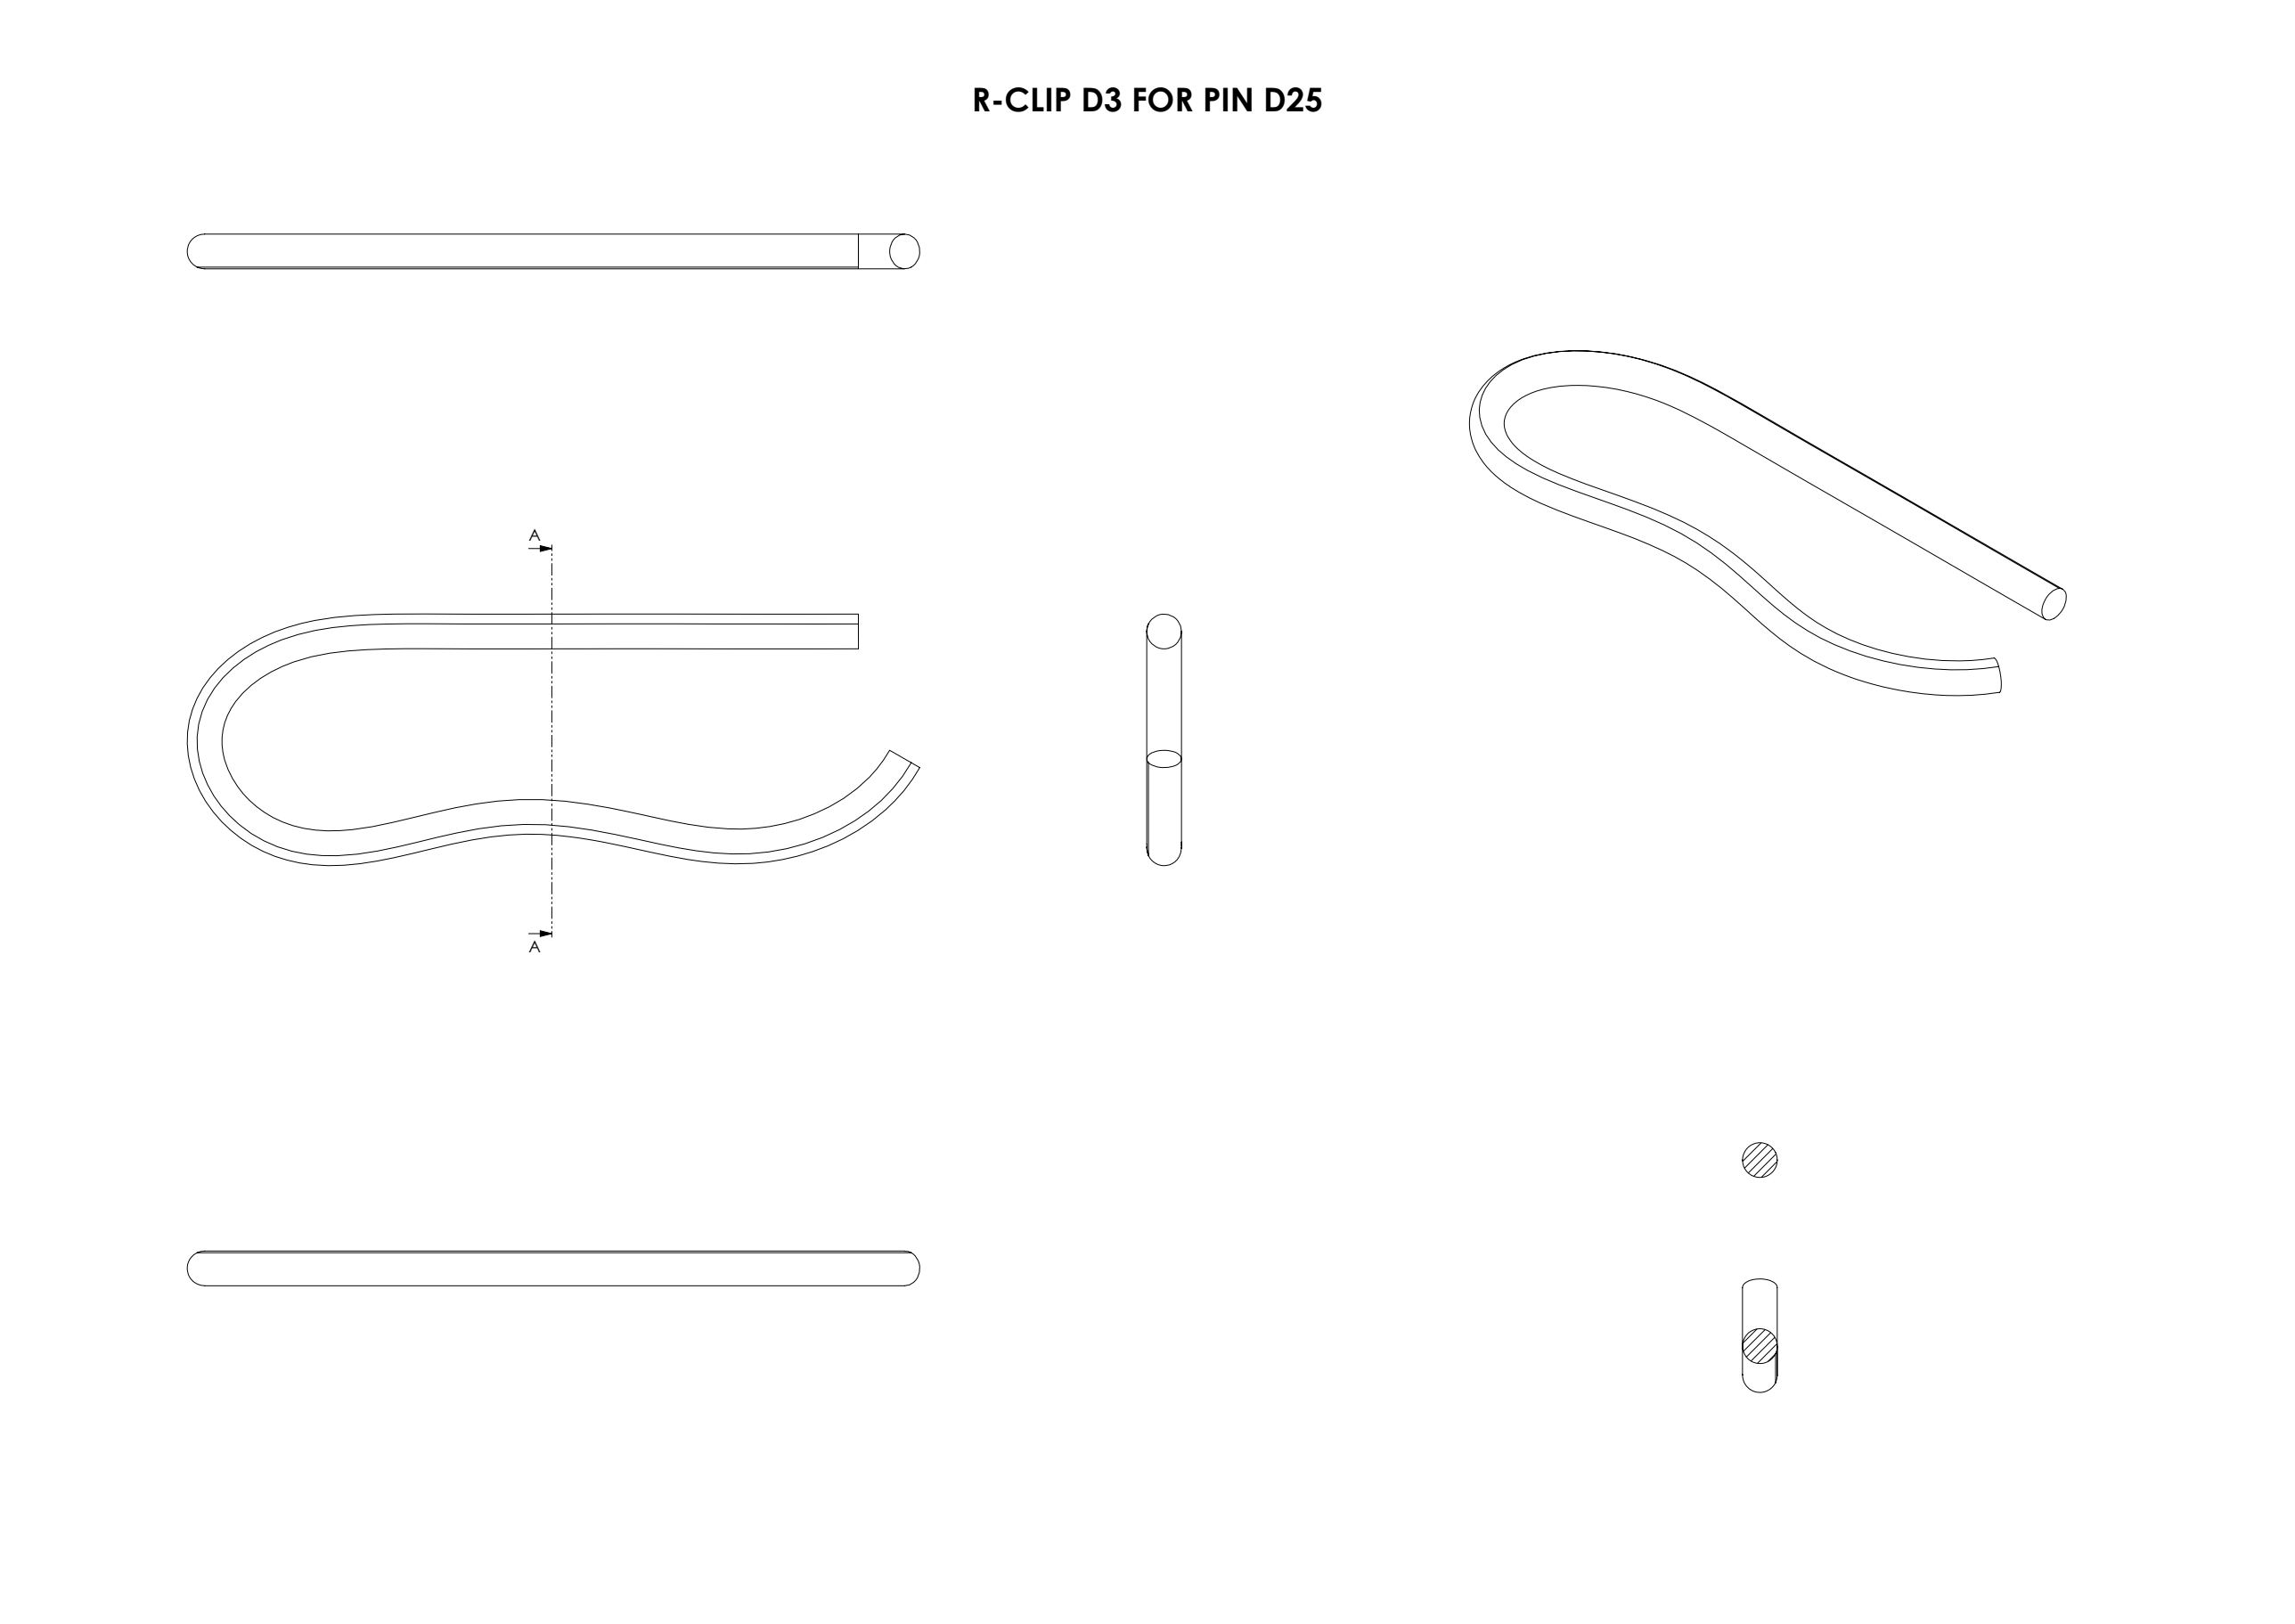
ISO-10303-21;
HEADER;
/* Generated by software containing ST-Developer
 * from STEP Tools, Inc. (www.steptools.com) 
 */

FILE_DESCRIPTION(
/* description */ (''),
/* implementation_level */ '2;1');

FILE_NAME(
/* name */ '06_R-Clip_D3_for_Pin_D25.step',
/* time_stamp */ '2026-10-20T10:03:03-07:00',
/* author */ (''),
/* organization */ (''),
/* preprocessor_version */ 'ST-DEVELOPER v20.2',
/* originating_system */ 'Autodesk Translation Framework v15.15.0.0',
/* authorisation */ '');

FILE_SCHEMA (('AUTOMOTIVE_DESIGN { 1 0 10303 214 3 1 1 }'));
ENDSEC;

DATA;
#10=MECHANICAL_DESIGN_GEOMETRIC_PRESENTATION_REPRESENTATION('',(#534),#71492);
#391=SHAPE_REPRESENTATION_RELATIONSHIP('SRR','None',#71612,#410);
#410=ADVANCED_BREP_SHAPE_REPRESENTATION('',(#429),#71482);
#429=MANIFOLD_SOLID_BREP('R-clip',#28468);
#534=STYLED_ITEM('',(#71887),#429);
#889=B_SPLINE_CURVE_WITH_KNOTS('',3,(#49969,#49970,#49971,#49972,#49973,
#49974,#49975,#49976,#49977,#49978,#49979,#49980,#49981,#49982,#49983,#49984,
#49985,#49986,#49987,#49988,#49989,#49990,#49991,#49992,#49993,#49994,#49995,
#49996,#49997,#49998),.UNSPECIFIED.,.F.,.F.,(4,1,1,1,1,1,1,1,1,1,1,1,1,
1,1,1,1,1,1,1,1,1,1,1,1,1,1,4),(0.,0.0714285714285714,0.142857142857143,
0.19047619047619,0.238095238095238,0.285714285714286,0.30952380952381,0.333333333333333,
0.357142857142857,0.380952380952381,0.404761904761905,0.428571428571429,
0.464285714285714,0.5,0.535714285714286,0.571428571428571,0.607142857142857,
0.642857142857143,0.678571428571428,0.714285714285714,0.767857142857143,
0.785714285714286,0.821428571428571,0.857142857142857,0.892857142857143,
0.928571428571429,0.964285714285714,1.),.UNSPECIFIED.);
#1460=B_SPLINE_SURFACE_WITH_KNOTS('',3,3,((#49636,#49637,#49638,#49639,
#49640,#49641,#49642,#49643,#49644,#49645,#49646,#49647,#49648,#49649,#49650,
#49651,#49652,#49653,#49654,#49655,#49656,#49657,#49658,#49659,#49660,#49661,
#49662,#49663,#49664,#49665),(#49666,#49667,#49668,#49669,#49670,#49671,
#49672,#49673,#49674,#49675,#49676,#49677,#49678,#49679,#49680,#49681,#49682,
#49683,#49684,#49685,#49686,#49687,#49688,#49689,#49690,#49691,#49692,#49693,
#49694,#49695),(#49696,#49697,#49698,#49699,#49700,#49701,#49702,#49703,
#49704,#49705,#49706,#49707,#49708,#49709,#49710,#49711,#49712,#49713,#49714,
#49715,#49716,#49717,#49718,#49719,#49720,#49721,#49722,#49723,#49724,#49725),
(#49726,#49727,#49728,#49729,#49730,#49731,#49732,#49733,#49734,#49735,
#49736,#49737,#49738,#49739,#49740,#49741,#49742,#49743,#49744,#49745,#49746,
#49747,#49748,#49749,#49750,#49751,#49752,#49753,#49754,#49755),(#49756,
#49757,#49758,#49759,#49760,#49761,#49762,#49763,#49764,#49765,#49766,#49767,
#49768,#49769,#49770,#49771,#49772,#49773,#49774,#49775,#49776,#49777,#49778,
#49779,#49780,#49781,#49782,#49783,#49784,#49785),(#49786,#49787,#49788,
#49789,#49790,#49791,#49792,#49793,#49794,#49795,#49796,#49797,#49798,#49799,
#49800,#49801,#49802,#49803,#49804,#49805,#49806,#49807,#49808,#49809,#49810,
#49811,#49812,#49813,#49814,#49815),(#49816,#49817,#49818,#49819,#49820,
#49821,#49822,#49823,#49824,#49825,#49826,#49827,#49828,#49829,#49830,#49831,
#49832,#49833,#49834,#49835,#49836,#49837,#49838,#49839,#49840,#49841,#49842,
#49843,#49844,#49845),(#49846,#49847,#49848,#49849,#49850,#49851,#49852,
#49853,#49854,#49855,#49856,#49857,#49858,#49859,#49860,#49861,#49862,#49863,
#49864,#49865,#49866,#49867,#49868,#49869,#49870,#49871,#49872,#49873,#49874,
#49875),(#49876,#49877,#49878,#49879,#49880,#49881,#49882,#49883,#49884,
#49885,#49886,#49887,#49888,#49889,#49890,#49891,#49892,#49893,#49894,#49895,
#49896,#49897,#49898,#49899,#49900,#49901,#49902,#49903,#49904,#49905),
(#49906,#49907,#49908,#49909,#49910,#49911,#49912,#49913,#49914,#49915,
#49916,#49917,#49918,#49919,#49920,#49921,#49922,#49923,#49924,#49925,#49926,
#49927,#49928,#49929,#49930,#49931,#49932,#49933,#49934,#49935),(#49936,
#49937,#49938,#49939,#49940,#49941,#49942,#49943,#49944,#49945,#49946,#49947,
#49948,#49949,#49950,#49951,#49952,#49953,#49954,#49955,#49956,#49957,#49958,
#49959,#49960,#49961,#49962,#49963,#49964,#49965)),.UNSPECIFIED.,.T.,.F.,
 .F.,(4,1,1,1,1,1,1,1,4),(4,1,1,1,1,1,1,1,1,1,1,1,1,1,1,1,1,1,1,1,1,1,1,
1,1,1,1,4),(-3.14159265358979,-2.69279370307697,-2.24399475256414,-1.34639685153848,
-0.448798950512828,0.448798950512828,1.34639685153848,2.24399475256414,
3.14159265358979),(0.,0.0714285714285714,0.142857142857143,0.19047619047619,
0.238095238095238,0.285714285714286,0.30952380952381,0.333333333333333,
0.357142857142857,0.380952380952381,0.404761904761905,0.428571428571429,
0.464285714285714,0.5,0.535714285714286,0.571428571428571,0.607142857142857,
0.642857142857143,0.678571428571428,0.714285714285714,0.767857142857143,
0.785714285714286,0.821428571428571,0.857142857142857,0.892857142857143,
0.928571428571429,0.964285714285714,1.),.UNSPECIFIED.);
#2477=CIRCLE('',#30009,0.15);
#2478=CIRCLE('',#30010,0.15);
#3961=FACE_OUTER_BOUND('',#5620,.T.);
#3962=FACE_OUTER_BOUND('',#5621,.T.);
#3963=FACE_OUTER_BOUND('',#5622,.T.);
#5620=EDGE_LOOP('',(#23039,#23040,#23041,#23042));
#5621=EDGE_LOOP('',(#23043));
#5622=EDGE_LOOP('',(#23044));
#12883=VERTEX_POINT('',#49966);
#12884=VERTEX_POINT('',#49968);
#16403=EDGE_CURVE('',#12883,#12883,#2477,.T.);
#16404=EDGE_CURVE('',#12883,#12884,#889,.T.);
#16405=EDGE_CURVE('',#12884,#12884,#2478,.T.);
#23039=ORIENTED_EDGE('',*,*,#16403,.T.);
#23040=ORIENTED_EDGE('',*,*,#16404,.T.);
#23041=ORIENTED_EDGE('',*,*,#16405,.F.);
#23042=ORIENTED_EDGE('',*,*,#16404,.F.);
#23043=ORIENTED_EDGE('',*,*,#16405,.T.);
#23044=ORIENTED_EDGE('',*,*,#16403,.F.);
#26673=PLANE('',#30011);
#26674=PLANE('',#30012);
#27869=ADVANCED_FACE('',(#3961),#1460,.T.);
#27870=ADVANCED_FACE('',(#3962),#26673,.T.);
#27871=ADVANCED_FACE('',(#3963),#26674,.F.);
#28468=CLOSED_SHELL('',(#27869,#27870,#27871));
#30008=AXIS2_PLACEMENT_3D('',#49635,#35201,#35202);
#30009=AXIS2_PLACEMENT_3D('',#49967,#35203,#35204);
#30010=AXIS2_PLACEMENT_3D('',#49999,#35205,#35206);
#30011=AXIS2_PLACEMENT_3D('',#50000,#35207,#35208);
#30012=AXIS2_PLACEMENT_3D('',#50001,#35209,#35210);
#35201=DIRECTION('axis',(0.,0.,1.));
#35202=DIRECTION('refdir',(1.,0.,0.));
#35203=DIRECTION('center_axis',(-0.99999684852218,9.62964972193618E-35,
0.00251056680999716));
#35204=DIRECTION('ref_axis',(3.0745576079086E-19,1.,1.22464293970013E-16));
#35205=DIRECTION('center_axis',(0.496743222852577,9.62964972193618E-35,
-0.867897557635712));
#35206=DIRECTION('ref_axis',(-1.06286796594638E-16,1.,-6.08334997864549E-17));
#35207=DIRECTION('center_axis',(0.496743222852577,9.62964972193618E-35,
-0.867897557635712));
#35208=DIRECTION('ref_axis',(-1.06286796594638E-16,1.,-6.08334997864549E-17));
#35209=DIRECTION('center_axis',(-0.99999684852218,9.62964972193618E-35,
0.00251056680999716));
#35210=DIRECTION('ref_axis',(3.0745576079086E-19,1.,1.22464293970013E-16));
#49635=CARTESIAN_POINT('',(0.,0.,0.));
#49636=CARTESIAN_POINT('Ctrl Pts',(32.6,10.85,74.75));
#49637=CARTESIAN_POINT('Ctrl Pts',(32.2762401972932,10.85,74.7508128231767));
#49638=CARTESIAN_POINT('Ctrl Pts',(31.6096093142576,10.85,74.7508592792408));
#49639=CARTESIAN_POINT('Ctrl Pts',(30.6649845099545,10.85,74.7480354284176));
#49640=CARTESIAN_POINT('Ctrl Pts',(29.7873935141465,10.85,74.7508112397276));
#49641=CARTESIAN_POINT('Ctrl Pts',(29.0359543531313,10.85,74.7503280524995));
#49642=CARTESIAN_POINT('Ctrl Pts',(28.4690072452371,10.85,74.7453827659742));
#49643=CARTESIAN_POINT('Ctrl Pts',(28.0559136155584,10.85,74.7762871198526));
#49644=CARTESIAN_POINT('Ctrl Pts',(27.7603250073182,10.85,74.8351351843659));
#49645=CARTESIAN_POINT('Ctrl Pts',(27.4815926484957,10.85,74.9426482833623));
#49646=CARTESIAN_POINT('Ctrl Pts',(27.2349066090381,10.85,75.1047310768146));
#49647=CARTESIAN_POINT('Ctrl Pts',(27.0488833547682,10.85,75.316337989367));
#49648=CARTESIAN_POINT('Ctrl Pts',(26.9333942799495,10.85,75.6052491869369));
#49649=CARTESIAN_POINT('Ctrl Pts',(26.9691269620806,10.85,75.9631669379198));
#49650=CARTESIAN_POINT('Ctrl Pts',(27.2040779638452,10.85,76.3230245921545));
#49651=CARTESIAN_POINT('Ctrl Pts',(27.5697532039707,10.85,76.564507863235));
#49652=CARTESIAN_POINT('Ctrl Pts',(28.0086353410587,10.85,76.644046754502));
#49653=CARTESIAN_POINT('Ctrl Pts',(28.4740751575422,10.85,76.5836894126618));
#49654=CARTESIAN_POINT('Ctrl Pts',(28.9373359185006,10.85,76.4628665594052));
#49655=CARTESIAN_POINT('Ctrl Pts',(29.391243866756,10.85,76.3646478753146));
#49656=CARTESIAN_POINT('Ctrl Pts',(29.9224229501769,10.85,76.3317150468999));
#49657=CARTESIAN_POINT('Ctrl Pts',(30.3862078321633,10.85,76.4084139727046));
#49658=CARTESIAN_POINT('Ctrl Pts',(30.8370751782289,10.85,76.5088290665611));
#49659=CARTESIAN_POINT('Ctrl Pts',(31.2017423456432,10.85,76.5874722844094));
#49660=CARTESIAN_POINT('Ctrl Pts',(31.6306430333322,10.85,76.6203631077507));
#49661=CARTESIAN_POINT('Ctrl Pts',(32.057764032766,10.85,76.5556313773306));
#49662=CARTESIAN_POINT('Ctrl Pts',(32.4547567135938,10.85,76.3953576871574));
#49663=CARTESIAN_POINT('Ctrl Pts',(32.7799571046759,10.85,76.160246076731));
#49664=CARTESIAN_POINT('Ctrl Pts',(32.936764346482,10.85,75.9604837805911));
#49665=CARTESIAN_POINT('Ctrl Pts',(33.,10.85,75.85));
#49666=CARTESIAN_POINT('Ctrl Pts',(32.6000563369875,10.85,74.7724398768066));
#49667=CARTESIAN_POINT('Ctrl Pts',(32.276260929417,10.85,74.773252789372));
#49668=CARTESIAN_POINT('Ctrl Pts',(31.6095450892366,10.85,74.7733264598551));
#49669=CARTESIAN_POINT('Ctrl Pts',(30.6649680305084,10.85,74.770524214627));
#49670=CARTESIAN_POINT('Ctrl Pts',(29.7874988197858,10.85,74.7733201933816));
#49671=CARTESIAN_POINT('Ctrl Pts',(29.0357590293253,10.85,74.772827717134));
#49672=CARTESIAN_POINT('Ctrl Pts',(28.4691172918998,10.85,74.7679357482136));
#49673=CARTESIAN_POINT('Ctrl Pts',(28.0587241075366,10.85,74.7986993033607));
#49674=CARTESIAN_POINT('Ctrl Pts',(27.7664700618278,10.85,74.8569322976131));
#49675=CARTESIAN_POINT('Ctrl Pts',(27.4918367913922,10.85,74.9629249524921));
#49676=CARTESIAN_POINT('Ctrl Pts',(27.2496218968497,10.85,75.1221404024895));
#49677=CARTESIAN_POINT('Ctrl Pts',(27.0682838610513,10.85,75.3287569874176));
#49678=CARTESIAN_POINT('Ctrl Pts',(26.9567767966594,10.85,75.6081224286654));
#49679=CARTESIAN_POINT('Ctrl Pts',(26.990989309624,10.85,75.9546108087208));
#49680=CARTESIAN_POINT('Ctrl Pts',(27.2204142671727,10.85,76.3066636425127));
#49681=CARTESIAN_POINT('Ctrl Pts',(27.5782958003512,10.85,76.542870690622));
#49682=CARTESIAN_POINT('Ctrl Pts',(28.008423773198,10.85,76.6211208212145));
#49683=CARTESIAN_POINT('Ctrl Pts',(28.4690883466175,10.85,76.5616816518995));
#49684=CARTESIAN_POINT('Ctrl Pts',(28.9315833093654,10.85,76.4410887479559));
#49685=CARTESIAN_POINT('Ctrl Pts',(29.3878485867094,10.85,76.3422677074518));
#49686=CARTESIAN_POINT('Ctrl Pts',(29.9240098885591,10.85,76.3090400645788));
#49687=CARTESIAN_POINT('Ctrl Pts',(30.3908025345374,10.85,76.3863518680965));
#49688=CARTESIAN_POINT('Ctrl Pts',(30.8421588378765,10.85,76.4868839589043));
#49689=CARTESIAN_POINT('Ctrl Pts',(31.2056042124841,10.85,76.5652084041602));
#49690=CARTESIAN_POINT('Ctrl Pts',(31.6300186898376,10.85,76.597644224807));
#49691=CARTESIAN_POINT('Ctrl Pts',(32.0517912777471,10.85,76.5337352307175));
#49692=CARTESIAN_POINT('Ctrl Pts',(32.4440368335229,10.85,76.3753717458181));
#49693=CARTESIAN_POINT('Ctrl Pts',(32.7643760861828,10.85,76.1436502815021));
#49694=CARTESIAN_POINT('Ctrl Pts',(32.9183725363797,10.85,75.9474433601901));
#49695=CARTESIAN_POINT('Ctrl Pts',(32.980524424349,10.85,75.8388531081455));
#49696=CARTESIAN_POINT('Ctrl Pts',(32.6001686447022,10.8603147982162,74.8171737433964));
#49697=CARTESIAN_POINT('Ctrl Pts',(32.2763031787803,10.8603147982162,74.8179868318485));
#49698=CARTESIAN_POINT('Ctrl Pts',(31.6094377488407,10.8603147982161,74.8180197771703));
#49699=CARTESIAN_POINT('Ctrl Pts',(30.6649729046424,10.8603147982162,74.8151630306089));
#49700=CARTESIAN_POINT('Ctrl Pts',(29.7877524648402,10.8603147982162,74.8179500966226));
#49701=CARTESIAN_POINT('Ctrl Pts',(29.0354254148949,10.8603147982162,74.8174167247621));
#49702=CARTESIAN_POINT('Ctrl Pts',(28.4693985677817,10.8603147982162,74.8125554634436));
#49703=CARTESIAN_POINT('Ctrl Pts',(28.0643229618056,10.8603147982162,74.8430210576306));
#49704=CARTESIAN_POINT('Ctrl Pts',(27.7786338309861,10.8603147982162,74.9000202289801));
#49705=CARTESIAN_POINT('Ctrl Pts',(27.5120694364702,10.8603147982162,75.0030004765062));
#49706=CARTESIAN_POINT('Ctrl Pts',(27.2786525998037,10.8603147982162,75.1565559636045));
#49707=CARTESIAN_POINT('Ctrl Pts',(27.106533890621,10.8603147982162,75.3533339117745));
#49708=CARTESIAN_POINT('Ctrl Pts',(27.0028575113137,10.8603147982162,75.6138882653673));
#49709=CARTESIAN_POINT('Ctrl Pts',(27.0340645306277,10.8603147982162,75.9378170546844));
#49710=CARTESIAN_POINT('Ctrl Pts',(27.2526034559054,10.8603147982162,76.274488465086));
#49711=CARTESIAN_POINT('Ctrl Pts',(27.5951158125273,10.8603147982162,76.5002428856615));
#49712=CARTESIAN_POINT('Ctrl Pts',(28.0079879414614,10.8603147982162,76.5759141203375));
#49713=CARTESIAN_POINT('Ctrl Pts',(28.4592263548061,10.8603147982162,76.5182386328934));
#49714=CARTESIAN_POINT('Ctrl Pts',(28.9201772975586,10.8603147982162,76.3980556836469));
#49715=CARTESIAN_POINT('Ctrl Pts',(29.3810653556096,10.8603147982161,76.2980313748935));
#49716=CARTESIAN_POINT('Ctrl Pts',(29.9269962160277,10.8603147982162,76.2641971595999));
#49717=CARTESIAN_POINT('Ctrl Pts',(30.3996417432911,10.8603147982161,76.3426700071549));
#49718=CARTESIAN_POINT('Ctrl Pts',(30.8519578972724,10.8603147982161,76.443435682308));
#49719=CARTESIAN_POINT('Ctrl Pts',(31.2129494545749,10.8603147982161,76.5211163903991));
#49720=CARTESIAN_POINT('Ctrl Pts',(31.6284955249479,10.8603147982162,76.5526529958711));
#49721=CARTESIAN_POINT('Ctrl Pts',(32.0396921756707,10.8603147982161,76.4903571871348));
#49722=CARTESIAN_POINT('Ctrl Pts',(32.4225403421799,10.8603147982161,76.3357529267033));
#49723=CARTESIAN_POINT('Ctrl Pts',(32.7332695950143,10.8603147982162,76.1107032847168));
#49724=CARTESIAN_POINT('Ctrl Pts',(32.8816804851804,10.8603147982162,75.9214962201899));
#49725=CARTESIAN_POINT('Ctrl Pts',(32.9416998884375,10.8603147982162,75.816631793055));
#49726=CARTESIAN_POINT('Ctrl Pts',(32.6003507870374,10.9173779978439,74.8897237988075));
#49727=CARTESIAN_POINT('Ctrl Pts',(32.2763706833012,10.9173779978439,74.8905371750664));
#49728=CARTESIAN_POINT('Ctrl Pts',(31.6092408059009,10.9173779978439,74.8906089842051));
#49729=CARTESIAN_POINT('Ctrl Pts',(30.6649391372427,10.9173779978439,74.8877716255048));
#49730=CARTESIAN_POINT('Ctrl Pts',(29.7881155384771,10.9173779978439,74.8905984912303));
#49731=CARTESIAN_POINT('Ctrl Pts',(29.0348227573495,10.9173779978439,74.8900235131441));
#49732=CARTESIAN_POINT('Ctrl Pts',(28.4697863721622,10.9173779978439,74.8852955412753));
#49733=CARTESIAN_POINT('Ctrl Pts',(28.073407529173,10.9173779978439,74.9152969842928));
#49734=CARTESIAN_POINT('Ctrl Pts',(27.7984566406093,10.9173779978439,74.9703036077729));
#49735=CARTESIAN_POINT('Ctrl Pts',(27.5450918599662,10.9173779978439,75.0683777464734));
#49736=CARTESIAN_POINT('Ctrl Pts',(27.3260710565629,10.9173779978439,75.2126918714373));
#49737=CARTESIAN_POINT('Ctrl Pts',(27.1690376611787,10.9173779978439,75.3933923333458));
#49738=CARTESIAN_POINT('Ctrl Pts',(27.0781798920543,10.9173779978439,75.6231973743156));
#49739=CARTESIAN_POINT('Ctrl Pts',(27.1044849838054,10.9173779978439,75.9102903143264));
#49740=CARTESIAN_POINT('Ctrl Pts',(27.3052250360147,10.9173779978439,76.2218198596427));
#49741=CARTESIAN_POINT('Ctrl Pts',(27.622626334009,10.9173779978439,76.4305496821952));
#49742=CARTESIAN_POINT('Ctrl Pts',(28.0072966464833,10.9173779978439,76.5020491981849));
#49743=CARTESIAN_POINT('Ctrl Pts',(28.4431445330614,10.9173779978439,76.4473077471168));
#49744=CARTESIAN_POINT('Ctrl Pts',(28.9016105836741,10.9173779978439,76.3278431856978));
#49745=CARTESIAN_POINT('Ctrl Pts',(29.3700804966718,10.9173779978439,76.2258701284851));
#49746=CARTESIAN_POINT('Ctrl Pts',(29.9320352589329,10.9173779978439,76.1910729980464));
#49747=CARTESIAN_POINT('Ctrl Pts',(30.4143311380162,10.9173779978439,76.2714959237099));
#49748=CARTESIAN_POINT('Ctrl Pts',(30.8682204343415,10.9173779978439,76.3726400416632));
#49749=CARTESIAN_POINT('Ctrl Pts',(31.2252524300623,10.9173779978439,76.449285856095));
#49750=CARTESIAN_POINT('Ctrl Pts',(31.6263329075708,10.9173779978439,76.4793554494757));
#49751=CARTESIAN_POINT('Ctrl Pts',(32.0202822219457,10.9173779978439,76.4197056854291));
#49752=CARTESIAN_POINT('Ctrl Pts',(32.3878166590065,10.9173779978439,76.2712520604576));
#49753=CARTESIAN_POINT('Ctrl Pts',(32.6828711573204,10.9173779978439,76.0571183509728));
#49754=CARTESIAN_POINT('Ctrl Pts',(32.8222036961853,10.9173779978439,75.8793607200281));
#49755=CARTESIAN_POINT('Ctrl Pts',(32.8787336741032,10.9173779978439,75.7805929311363));
#49756=CARTESIAN_POINT('Ctrl Pts',(32.6004197403532,11.0382323039103,74.9171889506208));
#49757=CARTESIAN_POINT('Ctrl Pts',(32.2763960824041,11.0382323039103,74.9180024362257));
#49758=CARTESIAN_POINT('Ctrl Pts',(31.6091627411914,11.0382323039103,74.91810506137));
#49759=CARTESIAN_POINT('Ctrl Pts',(30.6649199575373,11.0382323039103,74.9152915856771));
#49760=CARTESIAN_POINT('Ctrl Pts',(29.7882455741809,11.0382323039103,74.918141846035));
#49761=CARTESIAN_POINT('Ctrl Pts',(29.0345851556084,11.0382323039103,74.9175549113419));
#49762=CARTESIAN_POINT('Ctrl Pts',(28.4699226877837,11.0382323039103,74.9128902134163));
#49763=CARTESIAN_POINT('Ctrl Pts',(28.0768473126076,11.0382323039103,74.9427188731477));
#49764=CARTESIAN_POINT('Ctrl Pts',(27.8059755754844,11.0382323039104,74.9969724834831));
#49765=CARTESIAN_POINT('Ctrl Pts',(27.5576251549794,11.0382323039104,75.0931861718835));
#49766=CARTESIAN_POINT('Ctrl Pts',(27.3440737596402,11.0382323039103,75.2339923011634));
#49767=CARTESIAN_POINT('Ctrl Pts',(27.1927716423468,11.0382323039103,75.4085877577714));
#49768=CARTESIAN_POINT('Ctrl Pts',(27.1067848106127,11.0382323039103,75.6267150594627));
#49769=CARTESIAN_POINT('Ctrl Pts',(27.1312299556696,11.0382323039103,75.899824991557));
#49770=CARTESIAN_POINT('Ctrl Pts',(27.3252098550035,11.0382323039103,76.2018065323155));
#49771=CARTESIAN_POINT('Ctrl Pts',(27.6330764906777,11.0382323039103,76.4040802732469));
#49772=CARTESIAN_POINT('Ctrl Pts',(28.0070373299347,11.0382323039103,76.4740021623901));
#49773=CARTESIAN_POINT('Ctrl Pts',(28.4370430349808,11.0382323039103,76.4203827524898));
#49774=CARTESIAN_POINT('Ctrl Pts',(28.8945713347287,11.0382323039104,76.3011983644768));
#49775=CARTESIAN_POINT('Ctrl Pts',(29.3659244771377,11.0382323039103,76.198487991896));
#49776=CARTESIAN_POINT('Ctrl Pts',(29.933972930673,11.0382323039104,76.1633295300463));
#49777=CARTESIAN_POINT('Ctrl Pts',(30.4199463885132,11.0382323039103,76.2445009897536));
#49778=CARTESIAN_POINT('Ctrl Pts',(30.8744337504458,11.0382323039103,76.3457883146342));
#49779=CARTESIAN_POINT('Ctrl Pts',(31.2299698631872,11.0382323039103,76.4220437523547));
#49780=CARTESIAN_POINT('Ctrl Pts',(31.6255614351983,11.0382323039103,76.4515566535074));
#49781=CARTESIAN_POINT('Ctrl Pts',(32.0129668538595,11.0382323039103,76.3929131655577));
#49782=CARTESIAN_POINT('Ctrl Pts',(32.3746928081619,11.0382323039103,76.2467962447793));
#49783=CARTESIAN_POINT('Ctrl Pts',(32.663799662923,11.0382323039103,76.0368096155983));
#49784=CARTESIAN_POINT('Ctrl Pts',(32.7996924162414,11.0382323039103,75.8634012602469));
#49785=CARTESIAN_POINT('Ctrl Pts',(32.8548966608026,11.0382323039103,75.7669497601123));
#49786=CARTESIAN_POINT('Ctrl Pts',(32.6001868385096,11.1547886743356,74.8244206129357));
#49787=CARTESIAN_POINT('Ctrl Pts',(32.2763096092205,11.1547886743356,74.8252337309206));
#49788=CARTESIAN_POINT('Ctrl Pts',(31.6094110486143,11.1547886743356,74.8253028169753));
#49789=CARTESIAN_POINT('Ctrl Pts',(30.6649567181913,11.1547886743356,74.8224811471162));
#49790=CARTESIAN_POINT('Ctrl Pts',(29.7877738826518,11.1547886743356,74.825288870932));
#49791=CARTESIAN_POINT('Ctrl Pts',(29.0353462768564,11.1547886743356,74.8247589437306));
#49792=CARTESIAN_POINT('Ctrl Pts',(28.4694162812406,11.1547886743356,74.8199366672874));
#49793=CARTESIAN_POINT('Ctrl Pts',(28.0652317101301,11.1547886743356,74.8503617671289));
#49794=CARTESIAN_POINT('Ctrl Pts',(27.7806432308789,11.1547886743356,74.9071645160077));
#49795=CARTESIAN_POINT('Ctrl Pts',(27.5154321828776,11.1547886743356,75.0096483867191));
#49796=CARTESIAN_POINT('Ctrl Pts',(27.2834924502539,11.1547886743356,75.1622617256134));
#49797=CARTESIAN_POINT('Ctrl Pts',(27.1129215593886,11.1547886743356,75.3573965112237));
#49798=CARTESIAN_POINT('Ctrl Pts',(27.0105620979254,11.1547886743356,75.614805214542));
#49799=CARTESIAN_POINT('Ctrl Pts',(27.0412709960272,11.1547886743356,75.9349781814651));
#49800=CARTESIAN_POINT('Ctrl Pts',(27.2579878317068,11.1547886743356,76.269077945434));
#49801=CARTESIAN_POINT('Ctrl Pts',(27.5979349842812,11.1547886743356,76.493109562925));
#49802=CARTESIAN_POINT('Ctrl Pts',(28.0079236688243,11.1547886743356,76.5683674061805));
#49803=CARTESIAN_POINT('Ctrl Pts',(28.4575930727758,11.1547886743356,76.5110076457537));
#49804=CARTESIAN_POINT('Ctrl Pts',(28.9183017155932,11.1547886743356,76.3909129102924));
#49805=CARTESIAN_POINT('Ctrl Pts',(29.3799731095367,11.1547886743356,76.2906947846657));
#49806=CARTESIAN_POINT('Ctrl Pts',(29.927559751678,11.1547886743356,76.2567707916463));
#49807=CARTESIAN_POINT('Ctrl Pts',(30.4012178328891,11.1547886743356,76.3354590540619));
#49808=CARTESIAN_POINT('Ctrl Pts',(30.8536961803639,11.1547886743356,76.436262411816));
#49809=CARTESIAN_POINT('Ctrl Pts',(31.2142983985893,11.1547886743356,76.513842553578));
#49810=CARTESIAN_POINT('Ctrl Pts',(31.6283741100523,11.1547886743356,76.5452299621935));
#49811=CARTESIAN_POINT('Ctrl Pts',(32.0378187127339,11.1547886743356,76.4832076107804));
#49812=CARTESIAN_POINT('Ctrl Pts',(32.4191148073684,11.1547886743356,76.3292342878522));
#49813=CARTESIAN_POINT('Ctrl Pts',(32.7282509419986,11.1547886743356,76.1053043705975));
#49814=CARTESIAN_POINT('Ctrl Pts',(32.8757489865211,11.1547886743356,75.9172707791943));
#49815=CARTESIAN_POINT('Ctrl Pts',(32.9354103282424,11.1547886743356,75.8130319483797));
#49816=CARTESIAN_POINT('Ctrl Pts',(32.5998127104383,11.1547519764034,74.675399726197));
#49817=CARTESIAN_POINT('Ctrl Pts',(32.2761703317871,11.1547519764034,74.6762122545718));
#49818=CARTESIAN_POINT('Ctrl Pts',(31.6098016250815,11.1547519764034,74.6762655556816));
#49819=CARTESIAN_POINT('Ctrl Pts',(30.6650006393167,11.1547519764034,74.6734698551145));
#49820=CARTESIAN_POINT('Ctrl Pts',(29.7869986347378,11.1547519764034,74.6762289478734));
#49821=CARTESIAN_POINT('Ctrl Pts',(29.0365465597985,11.1547519764034,74.6757995710693));
#49822=CARTESIAN_POINT('Ctrl Pts',(28.4685779768367,11.1547519764034,74.6707544766575));
#49823=CARTESIAN_POINT('Ctrl Pts',(28.0465742254224,11.1547519764034,74.7021446137878));
#49824=CARTESIAN_POINT('Ctrl Pts',(27.7399845926101,11.1547519764034,74.7630453197478));
#49825=CARTESIAN_POINT('Ctrl Pts',(27.4477301966082,11.1547519764034,74.8755940064442));
#49826=CARTESIAN_POINT('Ctrl Pts',(27.1862980568975,11.1547519764034,75.0471516780439));
#49827=CARTESIAN_POINT('Ctrl Pts',(26.9848226471612,11.1547519764034,75.2752364149403));
#49828=CARTESIAN_POINT('Ctrl Pts',(26.8562056693994,11.1547519764034,75.5956582649194));
#49829=CARTESIAN_POINT('Ctrl Pts',(26.8969665026836,11.1547519764034,75.991342012992));
#49830=CARTESIAN_POINT('Ctrl Pts',(27.1501552309397,11.1547519764034,76.3769645604685));
#49831=CARTESIAN_POINT('Ctrl Pts',(27.5415685701483,11.1547519764034,76.6359212457116));
#49832=CARTESIAN_POINT('Ctrl Pts',(28.0093531063722,11.1547519764034,76.719754552362));
#49833=CARTESIAN_POINT('Ctrl Pts',(28.4905724048262,11.1547519764034,76.6564131286137));
#49834=CARTESIAN_POINT('Ctrl Pts',(28.9563968556498,11.1547519764034,76.5348754632395));
#49835=CARTESIAN_POINT('Ctrl Pts',(29.4025464173009,11.1547519764034,76.4386618160109));
#49836=CARTESIAN_POINT('Ctrl Pts',(29.9173288517,11.1547519764034,76.4067284088812));
#49837=CARTESIAN_POINT('Ctrl Pts',(30.3712611887102,11.1547519764034,76.4814520763918));
#49838=CARTESIAN_POINT('Ctrl Pts',(30.8205182721765,11.1547519764034,76.5814778598802));
#49839=CARTESIAN_POINT('Ctrl Pts',(31.1892658528984,11.1547519764034,76.6611892897302));
#49840=CARTESIAN_POINT('Ctrl Pts',(31.6330040350096,11.1547519764034,76.6955847221156));
#49841=CARTESIAN_POINT('Ctrl Pts',(32.0778173300849,11.1547519764034,76.6281454474494));
#49842=CARTESIAN_POINT('Ctrl Pts',(32.4905239707925,11.1547519764034,76.4615713425828));
#49843=CARTESIAN_POINT('Ctrl Pts',(32.8318023169732,11.1547519764034,76.215277917134));
#49844=CARTESIAN_POINT('Ctrl Pts',(32.9979357110749,11.1547519764034,76.0037858932076));
#49845=CARTESIAN_POINT('Ctrl Pts',(33.0647455994769,11.1547519764034,75.8870572972199));
#49846=CARTESIAN_POINT('Ctrl Pts',(32.5995793969032,11.0382369119409,74.5824674055347));
#49847=CARTESIAN_POINT('Ctrl Pts',(32.2760834569175,11.0382369119409,74.5832795662643));
#49848=CARTESIAN_POINT('Ctrl Pts',(31.6100447742661,11.0382369119409,74.5833249600566));
#49849=CARTESIAN_POINT('Ctrl Pts',(30.6650272601934,11.0382369119409,74.5805474438346));
#49850=CARTESIAN_POINT('Ctrl Pts',(29.7865142837032,11.0382369119409,74.5832772107547));
#49851=CARTESIAN_POINT('Ctrl Pts',(29.0372939426096,11.0382369119409,74.582910995395));
#49852=CARTESIAN_POINT('Ctrl Pts',(28.468053931887,11.0382369119409,74.5777284883834));
#49853=CARTESIAN_POINT('Ctrl Pts',(28.0349391340773,11.0382369119409,74.6097207938168));
#49854=CARTESIAN_POINT('Ctrl Pts',(27.7146308371164,11.0382369119409,74.6731772220513));
#49855=CARTESIAN_POINT('Ctrl Pts',(27.4055137767683,11.0382369119409,74.7920021444151));
#49856=CARTESIAN_POINT('Ctrl Pts',(27.1256919469879,11.0382369119409,74.9753727265389));
#49857=CARTESIAN_POINT('Ctrl Pts',(26.9049463387008,11.0382369119409,75.2240034592021));
#49858=CARTESIAN_POINT('Ctrl Pts',(26.7599568542985,11.0382369119409,75.583717079632));
#49859=CARTESIAN_POINT('Ctrl Pts',(26.8069857607438,11.0382369119409,76.0264862337433));
#49860=CARTESIAN_POINT('Ctrl Pts',(27.0829164167005,11.0382369119409,76.444235771622));
#49861=CARTESIAN_POINT('Ctrl Pts',(27.5064216534128,11.0382369119409,76.7249710719503));
#49862=CARTESIAN_POINT('Ctrl Pts',(28.0102448183053,11.0382369119409,76.8141524030629));
#49863=CARTESIAN_POINT('Ctrl Pts',(28.5111373421305,11.0382369119409,76.7470820576527));
#49864=CARTESIAN_POINT('Ctrl Pts',(28.9801524650468,11.0382369119409,76.6246455409694));
#49865=CARTESIAN_POINT('Ctrl Pts',(29.4166238712801,11.0382369119409,76.5309292146735));
#49866=CARTESIAN_POINT('Ctrl Pts',(29.910952277248,11.0382369119409,76.5002375601232));
#49867=CARTESIAN_POINT('Ctrl Pts',(30.3525861743777,11.0382369119409,76.5724900673701));
#49868=CARTESIAN_POINT('Ctrl Pts',(30.7998347185052,11.0382369119409,76.6720309332793));
#49869=CARTESIAN_POINT('Ctrl Pts',(31.1736622761221,11.0382369119409,76.7530716442971));
#49870=CARTESIAN_POINT('Ctrl Pts',(31.6358970252485,11.0382369119409,76.789342779067));
#49871=CARTESIAN_POINT('Ctrl Pts',(32.102765168382,11.0382369119409,76.7185259550485));
#49872=CARTESIAN_POINT('Ctrl Pts',(32.5350586903318,11.0382369119409,76.5440947520284));
#49873=CARTESIAN_POINT('Ctrl Pts',(32.8963798993568,11.0382369119409,76.2838567705243));
#49874=CARTESIAN_POINT('Ctrl Pts',(33.0741342976736,11.0382369119409,76.0577374019553));
#49875=CARTESIAN_POINT('Ctrl Pts',(33.1454015877907,11.0382369119409,75.9332209431765));
#49876=CARTESIAN_POINT('Ctrl Pts',(32.5996628076132,10.8930228127602,74.6156911567283));
#49877=CARTESIAN_POINT('Ctrl Pts',(32.2761145887457,10.8930228127602,74.6165034487079));
#49878=CARTESIAN_POINT('Ctrl Pts',(31.6099595038204,10.8930228127602,74.6165440657868));
#49879=CARTESIAN_POINT('Ctrl Pts',(30.6650207633387,10.8930228127602,74.6137522372086));
#49880=CARTESIAN_POINT('Ctrl Pts',(29.7866909415064,10.8930228127602,74.6164885561164));
#49881=CARTESIAN_POINT('Ctrl Pts',(29.0370312139308,10.8930228127602,74.6160979687152));
#49882=CARTESIAN_POINT('Ctrl Pts',(28.4682462358672,10.8930228127602,74.6109585365518));
#49883=CARTESIAN_POINT('Ctrl Pts',(28.03909842628,10.8930228127602,74.6427341806224));
#49884=CARTESIAN_POINT('Ctrl Pts',(27.723688010425,10.8930228127602,74.7052763109341));
#49885=CARTESIAN_POINT('Ctrl Pts',(27.4205912155809,10.8930228127602,74.8218589376446));
#49886=CARTESIAN_POINT('Ctrl Pts',(27.1473345686385,10.8930228127602,75.0010108373297));
#49887=CARTESIAN_POINT('Ctrl Pts',(26.9334684899571,10.8930228127602,75.2423050500824));
#49888=CARTESIAN_POINT('Ctrl Pts',(26.794323653363,10.8930228127602,75.5879891555652));
#49889=CARTESIAN_POINT('Ctrl Pts',(26.8391136919026,10.8930228127602,76.0139430513525));
#49890=CARTESIAN_POINT('Ctrl Pts',(27.1069244172984,10.8930228127602,76.4202212440923));
#49891=CARTESIAN_POINT('Ctrl Pts',(27.5189700615504,10.8930228127602,76.6931758299514));
#49892=CARTESIAN_POINT('Ctrl Pts',(28.0099249004793,10.8930228127602,76.7804444358118));
#49893=CARTESIAN_POINT('Ctrl Pts',(28.5037916195392,10.8930228127602,76.7147018584722));
#49894=CARTESIAN_POINT('Ctrl Pts',(28.9716646686748,10.8930228127602,76.5925828067522));
#49895=CARTESIAN_POINT('Ctrl Pts',(29.4115899334285,10.8930228127602,76.4979734783621));
#49896=CARTESIAN_POINT('Ctrl Pts',(29.9132177445037,10.8930228127602,76.4668363814021));
#49897=CARTESIAN_POINT('Ctrl Pts',(30.3592369373731,10.8930228127602,76.539967478678));
#49898=CARTESIAN_POINT('Ctrl Pts',(30.8072023523051,10.8930228127602,76.6396817330575));
#49899=CARTESIAN_POINT('Ctrl Pts',(31.1792123387399,10.8930228127602,76.7202465580442));
#49900=CARTESIAN_POINT('Ctrl Pts',(31.634840468396,10.8930228127602,76.7558477472188));
#49901=CARTESIAN_POINT('Ctrl Pts',(32.0938307914786,10.8930228127602,76.686236256697));
#49902=CARTESIAN_POINT('Ctrl Pts',(32.5191271929452,10.8930228127602,76.5146100998322));
#49903=CARTESIAN_POINT('Ctrl Pts',(32.8732894407117,10.8930228127602,76.259350444784));
#49904=CARTESIAN_POINT('Ctrl Pts',(33.046890695164,10.8930228127602,76.0384533948912));
#49905=CARTESIAN_POINT('Ctrl Pts',(33.1165666844017,10.8930228127602,75.9167172179222));
#49906=CARTESIAN_POINT('Ctrl Pts',(32.599887326025,10.85,74.7051202463867));
#49907=CARTESIAN_POINT('Ctrl Pts',(32.2761981190515,10.85,74.7059328923275));
#49908=CARTESIAN_POINT('Ctrl Pts',(31.6097239532025,10.85,74.7059883126997));
#49909=CARTESIAN_POINT('Ctrl Pts',(30.6649922884241,10.85,74.7031863758766));
#49910=CARTESIAN_POINT('Ctrl Pts',(29.7871537227045,10.85,74.7059546354782));
#49911=CARTESIAN_POINT('Ctrl Pts',(29.0363077810949,10.85,74.7055049626261));
#49912=CARTESIAN_POINT('Ctrl Pts',(28.4687458376382,10.85,74.7005034879709));
#49913=CARTESIAN_POINT('Ctrl Pts',(28.0502952066557,10.85,74.7317009722169));
#49914=CARTESIAN_POINT('Ctrl Pts',(27.7480925595316,10.85,74.791784304059));
#49915=CARTESIAN_POINT('Ctrl Pts',(27.4612305395664,10.85,74.9023258791797));
#49916=CARTESIAN_POINT('Ctrl Pts',(27.2056790773174,10.85,75.0701059267153));
#49917=CARTESIAN_POINT('Ctrl Pts',(27.0103659152346,10.85,75.29162035776));
#49918=CARTESIAN_POINT('Ctrl Pts',(26.8869845363635,10.85,75.599477318155));
#49919=CARTESIAN_POINT('Ctrl Pts',(26.9257408959584,10.85,75.9801037358516));
#49920=CARTESIAN_POINT('Ctrl Pts',(27.1716571299138,10.85,76.355452572985));
#49921=CARTESIAN_POINT('Ctrl Pts',(27.5528079390515,10.85,76.6074445605929));
#49922=CARTESIAN_POINT('Ctrl Pts',(28.0090678688855,10.85,76.6895674829939));
#49923=CARTESIAN_POINT('Ctrl Pts',(28.4839959103718,10.85,76.6274183114511));
#49924=CARTESIAN_POINT('Ctrl Pts',(28.9487998829859,10.85,76.5061678971924));
#49925=CARTESIAN_POINT('Ctrl Pts',(29.3980442681989,10.85,76.4091555755402));
#49926=CARTESIAN_POINT('Ctrl Pts',(29.9193673683687,10.85,76.3768249643973));
#49927=CARTESIAN_POINT('Ctrl Pts',(30.3772322305165,10.85,76.4523386674084));
#49928=CARTESIAN_POINT('Ctrl Pts',(30.8271315971887,10.85,76.5525195330394));
#49929=CARTESIAN_POINT('Ctrl Pts',(31.1942544811605,10.85,76.6318058122052));
#49930=CARTESIAN_POINT('Ctrl Pts',(31.6320776318315,10.85,76.665601413321));
#49931=CARTESIAN_POINT('Ctrl Pts',(32.0698379765199,10.85,76.599242190541));
#49932=CARTESIAN_POINT('Ctrl Pts',(32.4762808561744,10.85,76.435180639965));
#49933=CARTESIAN_POINT('Ctrl Pts',(32.8111496779181,10.85,76.193346425483));
#49934=CARTESIAN_POINT('Ctrl Pts',(32.9735666558701,10.85,75.9865319681108));
#49935=CARTESIAN_POINT('Ctrl Pts',(33.038951151302,10.85,75.8722937837091));
#49936=CARTESIAN_POINT('Ctrl Pts',(32.6,10.85,74.75));
#49937=CARTESIAN_POINT('Ctrl Pts',(32.2762401972932,10.85,74.7508128231767));
#49938=CARTESIAN_POINT('Ctrl Pts',(31.6096093142576,10.85,74.7508592792408));
#49939=CARTESIAN_POINT('Ctrl Pts',(30.6649845099545,10.85,74.7480354284176));
#49940=CARTESIAN_POINT('Ctrl Pts',(29.7873935141465,10.85,74.7508112397276));
#49941=CARTESIAN_POINT('Ctrl Pts',(29.0359543531313,10.85,74.7503280524995));
#49942=CARTESIAN_POINT('Ctrl Pts',(28.4690072452371,10.85,74.7453827659742));
#49943=CARTESIAN_POINT('Ctrl Pts',(28.0559136155584,10.85,74.7762871198526));
#49944=CARTESIAN_POINT('Ctrl Pts',(27.7603250073182,10.85,74.8351351843659));
#49945=CARTESIAN_POINT('Ctrl Pts',(27.4815926484957,10.85,74.9426482833623));
#49946=CARTESIAN_POINT('Ctrl Pts',(27.2349066090381,10.85,75.1047310768146));
#49947=CARTESIAN_POINT('Ctrl Pts',(27.0488833547682,10.85,75.316337989367));
#49948=CARTESIAN_POINT('Ctrl Pts',(26.9333942799495,10.85,75.6052491869369));
#49949=CARTESIAN_POINT('Ctrl Pts',(26.9691269620806,10.85,75.9631669379198));
#49950=CARTESIAN_POINT('Ctrl Pts',(27.2040779638452,10.85,76.3230245921545));
#49951=CARTESIAN_POINT('Ctrl Pts',(27.5697532039707,10.85,76.564507863235));
#49952=CARTESIAN_POINT('Ctrl Pts',(28.0086353410587,10.85,76.644046754502));
#49953=CARTESIAN_POINT('Ctrl Pts',(28.4740751575422,10.85,76.5836894126618));
#49954=CARTESIAN_POINT('Ctrl Pts',(28.9373359185006,10.85,76.4628665594052));
#49955=CARTESIAN_POINT('Ctrl Pts',(29.391243866756,10.85,76.3646478753146));
#49956=CARTESIAN_POINT('Ctrl Pts',(29.9224229501769,10.85,76.3317150468999));
#49957=CARTESIAN_POINT('Ctrl Pts',(30.3862078321633,10.85,76.4084139727046));
#49958=CARTESIAN_POINT('Ctrl Pts',(30.8370751782289,10.85,76.5088290665611));
#49959=CARTESIAN_POINT('Ctrl Pts',(31.2017423456432,10.85,76.5874722844094));
#49960=CARTESIAN_POINT('Ctrl Pts',(31.6306430333322,10.85,76.6203631077507));
#49961=CARTESIAN_POINT('Ctrl Pts',(32.057764032766,10.85,76.5556313773306));
#49962=CARTESIAN_POINT('Ctrl Pts',(32.4547567135938,10.85,76.3953576871574));
#49963=CARTESIAN_POINT('Ctrl Pts',(32.7799571046759,10.85,76.160246076731));
#49964=CARTESIAN_POINT('Ctrl Pts',(32.936764346482,10.85,75.9604837805911));
#49965=CARTESIAN_POINT('Ctrl Pts',(33.,10.85,75.85));
#49966=CARTESIAN_POINT('',(32.6,10.85,74.75));
#49967=CARTESIAN_POINT('Origin',(32.6,11.,74.75));
#49968=CARTESIAN_POINT('',(33.,10.85,75.85));
#49969=CARTESIAN_POINT('Ctrl Pts',(32.6,10.85,74.75));
#49970=CARTESIAN_POINT('Ctrl Pts',(32.2762401972932,10.85,74.7508128231767));
#49971=CARTESIAN_POINT('Ctrl Pts',(31.6096093142576,10.85,74.7508592792408));
#49972=CARTESIAN_POINT('Ctrl Pts',(30.6649845099545,10.85,74.7480354284176));
#49973=CARTESIAN_POINT('Ctrl Pts',(29.7873935141465,10.85,74.7508112397276));
#49974=CARTESIAN_POINT('Ctrl Pts',(29.0359543531313,10.85,74.7503280524995));
#49975=CARTESIAN_POINT('Ctrl Pts',(28.4690072452371,10.85,74.7453827659742));
#49976=CARTESIAN_POINT('Ctrl Pts',(28.0559136155584,10.85,74.7762871198526));
#49977=CARTESIAN_POINT('Ctrl Pts',(27.7603250073182,10.85,74.8351351843659));
#49978=CARTESIAN_POINT('Ctrl Pts',(27.4815926484957,10.85,74.9426482833623));
#49979=CARTESIAN_POINT('Ctrl Pts',(27.2349066090381,10.85,75.1047310768146));
#49980=CARTESIAN_POINT('Ctrl Pts',(27.0488833547682,10.85,75.316337989367));
#49981=CARTESIAN_POINT('Ctrl Pts',(26.9333942799495,10.85,75.6052491869369));
#49982=CARTESIAN_POINT('Ctrl Pts',(26.9691269620806,10.85,75.9631669379198));
#49983=CARTESIAN_POINT('Ctrl Pts',(27.2040779638452,10.85,76.3230245921545));
#49984=CARTESIAN_POINT('Ctrl Pts',(27.5697532039707,10.85,76.564507863235));
#49985=CARTESIAN_POINT('Ctrl Pts',(28.0086353410587,10.85,76.644046754502));
#49986=CARTESIAN_POINT('Ctrl Pts',(28.4740751575422,10.85,76.5836894126618));
#49987=CARTESIAN_POINT('Ctrl Pts',(28.9373359185006,10.85,76.4628665594052));
#49988=CARTESIAN_POINT('Ctrl Pts',(29.391243866756,10.85,76.3646478753146));
#49989=CARTESIAN_POINT('Ctrl Pts',(29.9224229501769,10.85,76.3317150468999));
#49990=CARTESIAN_POINT('Ctrl Pts',(30.3862078321633,10.85,76.4084139727046));
#49991=CARTESIAN_POINT('Ctrl Pts',(30.8370751782289,10.85,76.5088290665611));
#49992=CARTESIAN_POINT('Ctrl Pts',(31.2017423456432,10.85,76.5874722844094));
#49993=CARTESIAN_POINT('Ctrl Pts',(31.6306430333322,10.85,76.6203631077507));
#49994=CARTESIAN_POINT('Ctrl Pts',(32.057764032766,10.85,76.5556313773306));
#49995=CARTESIAN_POINT('Ctrl Pts',(32.4547567135938,10.85,76.3953576871574));
#49996=CARTESIAN_POINT('Ctrl Pts',(32.7799571046759,10.85,76.160246076731));
#49997=CARTESIAN_POINT('Ctrl Pts',(32.936764346482,10.85,75.9604837805911));
#49998=CARTESIAN_POINT('Ctrl Pts',(33.,10.85,75.85));
#49999=CARTESIAN_POINT('Origin',(33.,11.,75.85));
#50000=CARTESIAN_POINT('Origin',(33.,11.,75.85));
#50001=CARTESIAN_POINT('Origin',(32.6,11.,74.75));
#71461=UNCERTAINTY_MEASURE_WITH_UNIT(LENGTH_MEASURE(0.001),#71493,
'DISTANCE_ACCURACY_VALUE',
'Maximum model space distance between geometric entities at asserted c
onnectivities');
#71471=UNCERTAINTY_MEASURE_WITH_UNIT(LENGTH_MEASURE(0.001),#71493,
'DISTANCE_ACCURACY_VALUE',
'Maximum model space distance between geometric entities at asserted c
onnectivities');
#71482=(
GEOMETRIC_REPRESENTATION_CONTEXT(3)
GLOBAL_UNCERTAINTY_ASSIGNED_CONTEXT((#71461))
GLOBAL_UNIT_ASSIGNED_CONTEXT((#71493,#71495,#71496))
REPRESENTATION_CONTEXT('','3D')
);
#71492=(
GEOMETRIC_REPRESENTATION_CONTEXT(3)
GLOBAL_UNCERTAINTY_ASSIGNED_CONTEXT((#71471))
GLOBAL_UNIT_ASSIGNED_CONTEXT((#71493,#71495,#71496))
REPRESENTATION_CONTEXT('','3D')
);
#71493=(
LENGTH_UNIT()
NAMED_UNIT(*)
SI_UNIT(.CENTI.,.METRE.)
);
#71495=(
NAMED_UNIT(*)
PLANE_ANGLE_UNIT()
SI_UNIT($,.RADIAN.)
);
#71496=(
NAMED_UNIT(*)
SI_UNIT($,.STERADIAN.)
SOLID_ANGLE_UNIT()
);
#71507=SHAPE_DEFINITION_REPRESENTATION(#71527,#71612);
#71527=PRODUCT_DEFINITION_SHAPE('',$,#71633);
#71612=SHAPE_REPRESENTATION('',(#30008),#71482);
#71622=PRODUCT_DEFINITION_CONTEXT('part definition',#71684,'design');
#71633=PRODUCT_DEFINITION('2026-10-19-03-21-54-863',
'06_R-Clip_D3_for_Pin_D25',#71653,#71622);
#71653=PRODUCT_DEFINITION_FORMATION('',$,#71696);
#71684=APPLICATION_CONTEXT(
'Core Data for Automotive Mechanical Design Process');
#71685=PRODUCT_CONTEXT('part definition',#71684,'mechanical');
#71696=PRODUCT('2026-10-19-03-21-54-863','06_R-Clip_D3_for_Pin_D25',$,(#71685));
#71881=COLOUR_RGB('Grey',0.48,0.52,0.57);
#71882=FILL_AREA_STYLE_COLOUR('',#71881);
#71883=FILL_AREA_STYLE('',(#71882));
#71884=SURFACE_STYLE_FILL_AREA(#71883);
#71885=SURFACE_SIDE_STYLE('',(#71884));
#71886=SURFACE_STYLE_USAGE(.BOTH.,#71885);
#71887=PRESENTATION_STYLE_ASSIGNMENT((#71886));
ENDSEC;
END-ISO-10303-21;
